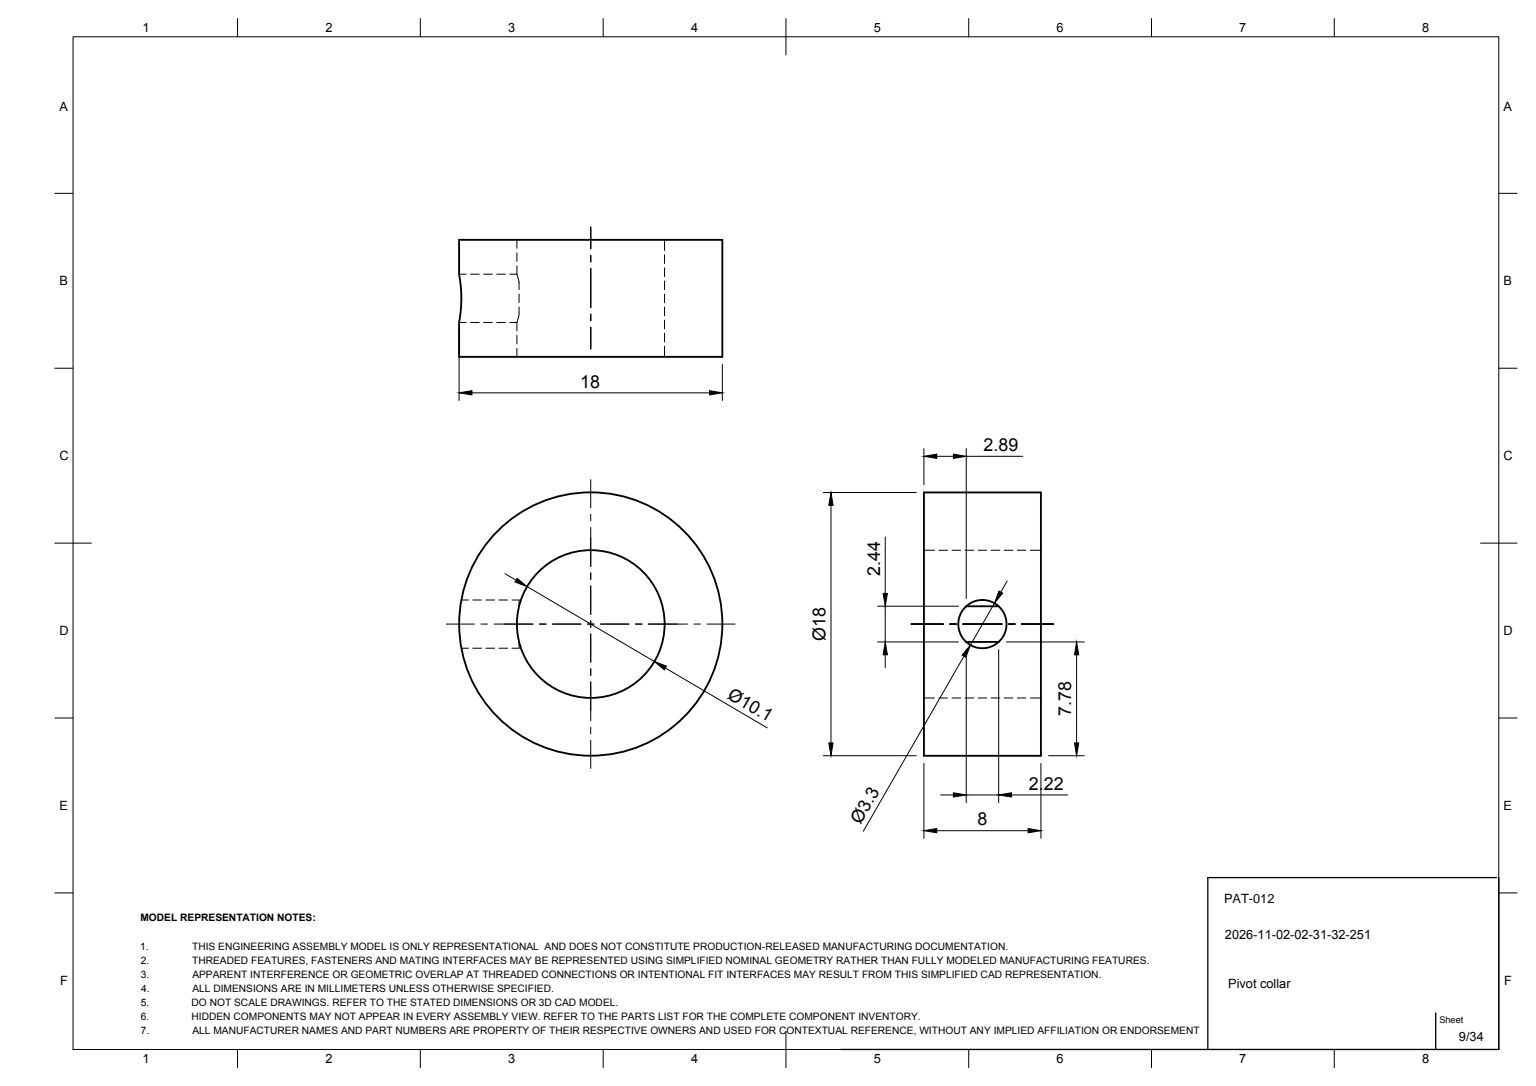
ISO-10303-21;
HEADER;
/* Generated by software containing ST-Developer
 * from STEP Tools, Inc. (www.steptools.com) 
 */

FILE_DESCRIPTION(
/* description */ ('Belt tensioner idler arm'),
/* implementation_level */ '2;1');

FILE_NAME(
/* name */ 'Pivot collar.step',
/* time_stamp */ '2026-10-28T03:22:15-07:00',
/* author */ (''),
/* organization */ (''),
/* preprocessor_version */ 'ST-DEVELOPER v20.2',
/* originating_system */ 'Autodesk Translation Framework v15.17.0.0',
/* authorisation */ '');

FILE_SCHEMA (('AUTOMOTIVE_DESIGN { 1 0 10303 214 3 1 1 }'));
ENDSEC;

DATA;
#10=MECHANICAL_DESIGN_GEOMETRIC_PRESENTATION_REPRESENTATION('',(#451),#12779);
#317=B_SPLINE_CURVE_WITH_KNOTS('',3,(#9613,#9614,#9615,#9616,#9617,#9618,
#9619,#9620,#9621,#9622,#9623,#9624,#9625,#9626),.UNSPECIFIED.,.F.,.F.,
(4,2,2,2,2,2,4),(0.618551524396292,0.626563103102765,0.689203386094988,
0.751843669087211,0.814483952079434,0.877124235071657,0.88513581377813),
 .UNSPECIFIED.);
#318=B_SPLINE_CURVE_WITH_KNOTS('',3,(#9630,#9631,#9632,#9633,#9634,#9635,
#9636,#9637),.UNSPECIFIED.,.F.,.F.,(4,2,2,4),(0.250614556362404,0.313254839354627,
0.37589512234685,0.383906701053323),.UNSPECIFIED.);
#319=B_SPLINE_CURVE_WITH_KNOTS('',3,(#9641,#9642,#9643,#9644,#9645,#9646,
#9647,#9648,#9649,#9650,#9651,#9652,#9653,#9654,#9655,#9656,#9657,#9658,
#9659,#9660,#9661,#9662,#9663,#9664,#9665,#9666),.UNSPECIFIED.,.F.,.F.,
(4,2,2,2,2,2,2,2,2,2,2,2,4),(0.,0.0623062782223143,0.124612556444629,0.186916384615149,
0.249220212785669,0.31152404095619,0.37382786912671,0.436134147349024,0.498440425571339,
0.560746703793653,0.623052982015967,0.685356810186488,0.747660638357008),
 .UNSPECIFIED.);
#320=B_SPLINE_CURVE_WITH_KNOTS('',3,(#9667,#9668,#9669,#9670,#9671,#9672,
#9673,#9674,#9675,#9676),.UNSPECIFIED.,.F.,.F.,(4,2,2,2,4),(0.747660638357008,
0.809964466527528,0.872268294698049,0.934574572920363,0.996880851142677),
 .UNSPECIFIED.);
#321=B_SPLINE_CURVE_WITH_KNOTS('',3,(#9677,#9678,#9679,#9680,#9681,#9682,
#9683,#9684),.UNSPECIFIED.,.F.,.F.,(4,2,2,4),(0.117322411671484,0.125333990377958,
0.187974273370181,0.250614556362404),.UNSPECIFIED.);
#383=SHAPE_REPRESENTATION_RELATIONSHIP('SRR','None',#12929,#417);
#417=ADVANCED_BREP_SHAPE_REPRESENTATION('',(#493),#12746);
#451=STYLED_ITEM('',(#13170),#493);
#493=MANIFOLD_SOLID_BREP('Body1',#6185);
#546=FACE_BOUND('',#1262,.T.);
#547=FACE_BOUND('',#1264,.T.);
#548=FACE_BOUND('',#1266,.T.);
#549=FACE_BOUND('',#1268,.T.);
#686=PLANE('',#6668);
#687=PLANE('',#6672);
#688=PLANE('',#6679);
#689=PLANE('',#6680);
#872=FACE_OUTER_BOUND('',#1258,.T.);
#873=FACE_OUTER_BOUND('',#1259,.T.);
#874=FACE_OUTER_BOUND('',#1260,.T.);
#875=FACE_OUTER_BOUND('',#1261,.T.);
#876=FACE_OUTER_BOUND('',#1263,.T.);
#877=FACE_OUTER_BOUND('',#1265,.T.);
#878=FACE_OUTER_BOUND('',#1267,.T.);
#1258=EDGE_LOOP('',(#4230,#4231));
#1259=EDGE_LOOP('',(#4232,#4233,#4234,#4235,#4236,#4237,#4238,#4239,#4240));
#1260=EDGE_LOOP('',(#4241,#4242));
#1261=EDGE_LOOP('',(#4243,#4244,#4245,#4246));
#1262=EDGE_LOOP('',(#4247,#4248,#4249,#4250,#4251));
#1263=EDGE_LOOP('',(#4252,#4253,#4254,#4255));
#1264=EDGE_LOOP('',(#4256,#4257));
#1265=EDGE_LOOP('',(#4258));
#1266=EDGE_LOOP('',(#4259));
#1267=EDGE_LOOP('',(#4260));
#1268=EDGE_LOOP('',(#4261));
#1755=LINE('',#9609,#2104);
#1756=LINE('',#9639,#2105);
#1757=LINE('',#9686,#2106);
#1758=LINE('',#9691,#2107);
#1759=LINE('',#9697,#2108);
#2104=VECTOR('',#7615,1.);
#2105=VECTOR('',#7622,0.165);
#2106=VECTOR('',#7625,1.);
#2107=VECTOR('',#7630,0.505);
#2108=VECTOR('',#7637,0.9);
#2429=CIRCLE('',#6669,0.165);
#2430=CIRCLE('',#6671,0.165);
#2431=CIRCLE('',#6674,0.505);
#2432=CIRCLE('',#6675,0.505);
#2433=CIRCLE('',#6677,0.9);
#2434=CIRCLE('',#6678,0.9);
#2817=VERTEX_POINT('',#9607);
#2818=VERTEX_POINT('',#9608);
#2819=VERTEX_POINT('',#9612);
#2820=VERTEX_POINT('',#9627);
#2821=VERTEX_POINT('',#9629);
#2822=VERTEX_POINT('',#9638);
#2823=VERTEX_POINT('',#9640);
#2824=VERTEX_POINT('',#9688);
#2825=VERTEX_POINT('',#9690);
#2826=VERTEX_POINT('',#9694);
#2827=VERTEX_POINT('',#9696);
#3370=EDGE_CURVE('',#2817,#2818,#1755,.T.);
#3371=EDGE_CURVE('',#2817,#2818,#2429,.T.);
#3372=EDGE_CURVE('',#2819,#2817,#317,.T.);
#3373=EDGE_CURVE('',#2820,#2819,#2430,.T.);
#3374=EDGE_CURVE('',#2821,#2820,#318,.T.);
#3375=EDGE_CURVE('',#2821,#2822,#1756,.T.);
#3376=EDGE_CURVE('',#2823,#2822,#319,.T.);
#3377=EDGE_CURVE('',#2822,#2823,#320,.T.);
#3378=EDGE_CURVE('',#2818,#2821,#321,.T.);
#3379=EDGE_CURVE('',#2820,#2819,#1757,.T.);
#3380=EDGE_CURVE('',#2824,#2824,#2431,.T.);
#3381=EDGE_CURVE('',#2824,#2825,#1758,.T.);
#3382=EDGE_CURVE('',#2825,#2825,#2432,.T.);
#3383=EDGE_CURVE('',#2826,#2826,#2433,.T.);
#3384=EDGE_CURVE('',#2826,#2827,#1759,.T.);
#3385=EDGE_CURVE('',#2827,#2827,#2434,.T.);
#4230=ORIENTED_EDGE('',*,*,#3370,.F.);
#4231=ORIENTED_EDGE('',*,*,#3371,.T.);
#4232=ORIENTED_EDGE('',*,*,#3372,.F.);
#4233=ORIENTED_EDGE('',*,*,#3373,.F.);
#4234=ORIENTED_EDGE('',*,*,#3374,.F.);
#4235=ORIENTED_EDGE('',*,*,#3375,.T.);
#4236=ORIENTED_EDGE('',*,*,#3376,.F.);
#4237=ORIENTED_EDGE('',*,*,#3377,.F.);
#4238=ORIENTED_EDGE('',*,*,#3375,.F.);
#4239=ORIENTED_EDGE('',*,*,#3378,.F.);
#4240=ORIENTED_EDGE('',*,*,#3371,.F.);
#4241=ORIENTED_EDGE('',*,*,#3379,.F.);
#4242=ORIENTED_EDGE('',*,*,#3373,.T.);
#4243=ORIENTED_EDGE('',*,*,#3380,.F.);
#4244=ORIENTED_EDGE('',*,*,#3381,.T.);
#4245=ORIENTED_EDGE('',*,*,#3382,.T.);
#4246=ORIENTED_EDGE('',*,*,#3381,.F.);
#4247=ORIENTED_EDGE('',*,*,#3378,.T.);
#4248=ORIENTED_EDGE('',*,*,#3374,.T.);
#4249=ORIENTED_EDGE('',*,*,#3379,.T.);
#4250=ORIENTED_EDGE('',*,*,#3372,.T.);
#4251=ORIENTED_EDGE('',*,*,#3370,.T.);
#4252=ORIENTED_EDGE('',*,*,#3383,.F.);
#4253=ORIENTED_EDGE('',*,*,#3384,.T.);
#4254=ORIENTED_EDGE('',*,*,#3385,.T.);
#4255=ORIENTED_EDGE('',*,*,#3384,.F.);
#4256=ORIENTED_EDGE('',*,*,#3376,.T.);
#4257=ORIENTED_EDGE('',*,*,#3377,.T.);
#4258=ORIENTED_EDGE('',*,*,#3383,.T.);
#4259=ORIENTED_EDGE('',*,*,#3380,.T.);
#4260=ORIENTED_EDGE('',*,*,#3385,.F.);
#4261=ORIENTED_EDGE('',*,*,#3382,.F.);
#5674=CYLINDRICAL_SURFACE('',#6670,0.165);
#5675=CYLINDRICAL_SURFACE('',#6673,0.505);
#5676=CYLINDRICAL_SURFACE('',#6676,0.9);
#5849=ADVANCED_FACE('',(#872),#686,.T.);
#5850=ADVANCED_FACE('',(#873),#5674,.F.);
#5851=ADVANCED_FACE('',(#874),#687,.T.);
#5852=ADVANCED_FACE('',(#875,#546),#5675,.F.);
#5853=ADVANCED_FACE('',(#876,#547),#5676,.T.);
#5854=ADVANCED_FACE('',(#877,#548),#688,.T.);
#5855=ADVANCED_FACE('',(#878,#549),#689,.F.);
#6185=CLOSED_SHELL('',(#5849,#5850,#5851,#5852,#5853,#5854,#5855));
#6667=AXIS2_PLACEMENT_3D('',#9605,#7611,#7612);
#6668=AXIS2_PLACEMENT_3D('',#9606,#7613,#7614);
#6669=AXIS2_PLACEMENT_3D('',#9610,#7616,#7617);
#6670=AXIS2_PLACEMENT_3D('',#9611,#7618,#7619);
#6671=AXIS2_PLACEMENT_3D('',#9628,#7620,#7621);
#6672=AXIS2_PLACEMENT_3D('',#9685,#7623,#7624);
#6673=AXIS2_PLACEMENT_3D('',#9687,#7626,#7627);
#6674=AXIS2_PLACEMENT_3D('',#9689,#7628,#7629);
#6675=AXIS2_PLACEMENT_3D('',#9692,#7631,#7632);
#6676=AXIS2_PLACEMENT_3D('',#9693,#7633,#7634);
#6677=AXIS2_PLACEMENT_3D('',#9695,#7635,#7636);
#6678=AXIS2_PLACEMENT_3D('',#9698,#7638,#7639);
#6679=AXIS2_PLACEMENT_3D('',#9699,#7640,#7641);
#6680=AXIS2_PLACEMENT_3D('',#9700,#7642,#7643);
#7611=DIRECTION('axis',(0.,0.,1.));
#7612=DIRECTION('refdir',(1.,0.,0.));
#7613=DIRECTION('center_axis',(1.,0.,0.));
#7614=DIRECTION('ref_axis',(0.,0.,-1.));
#7615=DIRECTION('',(0.,0.,1.));
#7616=DIRECTION('center_axis',(1.,0.,0.));
#7617=DIRECTION('ref_axis',(0.,0.,-1.));
#7618=DIRECTION('center_axis',(1.,0.,0.));
#7619=DIRECTION('ref_axis',(0.,0.,-1.));
#7620=DIRECTION('center_axis',(1.,0.,0.));
#7621=DIRECTION('ref_axis',(0.,0.,-1.));
#7622=DIRECTION('',(1.,0.,0.));
#7623=DIRECTION('center_axis',(1.,0.,0.));
#7624=DIRECTION('ref_axis',(0.,0.,-1.));
#7625=DIRECTION('',(0.,0.,-1.));
#7626=DIRECTION('center_axis',(0.,0.,1.));
#7627=DIRECTION('ref_axis',(1.,0.,0.));
#7628=DIRECTION('center_axis',(0.,0.,-1.));
#7629=DIRECTION('ref_axis',(1.,0.,0.));
#7630=DIRECTION('',(0.,0.,-1.));
#7631=DIRECTION('center_axis',(0.,0.,-1.));
#7632=DIRECTION('ref_axis',(1.,0.,0.));
#7633=DIRECTION('center_axis',(0.,0.,1.));
#7634=DIRECTION('ref_axis',(1.,0.,0.));
#7635=DIRECTION('center_axis',(0.,0.,1.));
#7636=DIRECTION('ref_axis',(1.,0.,0.));
#7637=DIRECTION('',(0.,0.,-1.));
#7638=DIRECTION('center_axis',(0.,0.,1.));
#7639=DIRECTION('ref_axis',(1.,0.,0.));
#7640=DIRECTION('center_axis',(0.,0.,1.));
#7641=DIRECTION('ref_axis',(1.,0.,0.));
#7642=DIRECTION('center_axis',(0.,0.,1.));
#7643=DIRECTION('ref_axis',(1.,0.,0.));
#9605=CARTESIAN_POINT('',(0.,0.,0.));
#9606=CARTESIAN_POINT('Origin',(0.49,0.,6.35));
#9607=CARTESIAN_POINT('',(0.49,0.122167917228706,6.2390946349359));
#9608=CARTESIAN_POINT('',(0.49,0.122167917228706,6.46090536506409));
#9609=CARTESIAN_POINT('',(0.49,0.122167917228706,5.95));
#9610=CARTESIAN_POINT('Origin',(0.49,0.,6.35));
#9611=CARTESIAN_POINT('Origin',(0.49,0.,6.35));
#9612=CARTESIAN_POINT('',(0.49,-0.122167917228706,6.2390946349359));
#9613=CARTESIAN_POINT('Ctrl Pts',(0.49,-0.122167917228706,6.2390946349359));
#9614=CARTESIAN_POINT('Ctrl Pts',(0.490448531679987,-0.120368913626295,
6.23711294069536));
#9615=CARTESIAN_POINT('Ctrl Pts',(0.490895245371684,-0.118534896565231,
6.23518965877367));
#9616=CARTESIAN_POINT('Ctrl Pts',(0.494795015531646,-0.102111993019358,
6.2187667552278));
#9617=CARTESIAN_POINT('Ctrl Pts',(0.498442514607595,-0.0836597150224318,
6.20609154388858));
#9618=CARTESIAN_POINT('Ctrl Pts',(0.50357781976106,-0.0430495960471596,
6.18920409039234));
#9619=CARTESIAN_POINT('Ctrl Pts',(0.505,-0.020880094330741,6.185));
#9620=CARTESIAN_POINT('Ctrl Pts',(0.505,0.020880094330741,6.185));
#9621=CARTESIAN_POINT('Ctrl Pts',(0.50357781976106,0.0430495960471596,6.18920409039234));
#9622=CARTESIAN_POINT('Ctrl Pts',(0.498442514607595,0.0836597150224318,
6.20609154388858));
#9623=CARTESIAN_POINT('Ctrl Pts',(0.494795015531646,0.102111993019358,6.2187667552278));
#9624=CARTESIAN_POINT('Ctrl Pts',(0.490895245371685,0.118534896565231,6.23518965877367));
#9625=CARTESIAN_POINT('Ctrl Pts',(0.490448531679987,0.120368913626295,6.23711294069536));
#9626=CARTESIAN_POINT('Ctrl Pts',(0.49,0.122167917228706,6.2390946349359));
#9627=CARTESIAN_POINT('',(0.49,-0.122167917228706,6.46090536506409));
#9628=CARTESIAN_POINT('Origin',(0.49,0.,6.35));
#9629=CARTESIAN_POINT('',(0.505,4.88772620902458E-17,6.515));
#9630=CARTESIAN_POINT('Ctrl Pts',(0.505,1.2490009027033E-16,6.515));
#9631=CARTESIAN_POINT('Ctrl Pts',(0.505,-0.0208800943307409,6.515));
#9632=CARTESIAN_POINT('Ctrl Pts',(0.50357781976106,-0.0430495960471596,
6.51079590960766));
#9633=CARTESIAN_POINT('Ctrl Pts',(0.498442514607595,-0.0836597150224318,
6.49390845611142));
#9634=CARTESIAN_POINT('Ctrl Pts',(0.494795015531646,-0.102111993019358,
6.4812332447722));
#9635=CARTESIAN_POINT('Ctrl Pts',(0.490895245371684,-0.118534896565231,
6.46481034122633));
#9636=CARTESIAN_POINT('Ctrl Pts',(0.490448531679987,-0.120368913626296,
6.46288705930464));
#9637=CARTESIAN_POINT('Ctrl Pts',(0.49,-0.122167917228706,6.46090536506409));
#9638=CARTESIAN_POINT('',(0.9,-2.02066721859313E-17,6.515));
#9639=CARTESIAN_POINT('',(0.49,-2.02066721859313E-17,6.515));
#9640=CARTESIAN_POINT('',(0.884745726183518,0.165,6.35));
#9641=CARTESIAN_POINT('Ctrl Pts',(0.884745726183518,0.165,6.35));
#9642=CARTESIAN_POINT('Ctrl Pts',(0.884745726183518,0.165,6.32923124059256));
#9643=CARTESIAN_POINT('Ctrl Pts',(0.885552759505264,0.160839719007584,6.30711110492665));
#9644=CARTESIAN_POINT('Ctrl Pts',(0.888448648150043,0.14398647021669,6.26647293736623));
#9645=CARTESIAN_POINT('Ctrl Pts',(0.890493604851638,0.131295993814186,6.24795075602263));
#9646=CARTESIAN_POINT('Ctrl Pts',(0.89431723432394,0.102049819008125,6.21870458121656));
#9647=CARTESIAN_POINT('Ctrl Pts',(0.896347088899543,0.0835273920906821,
6.20601365401642));
#9648=CARTESIAN_POINT('Ctrl Pts',(0.899208271860583,0.0428883760934128,
6.18916007816136));
#9649=CARTESIAN_POINT('Ctrl Pts',(0.9,0.0207679427235068,6.185));
#9650=CARTESIAN_POINT('Ctrl Pts',(0.9,-0.0207679427235068,6.185));
#9651=CARTESIAN_POINT('Ctrl Pts',(0.899208271860583,-0.0428883760934128,
6.18916007816136));
#9652=CARTESIAN_POINT('Ctrl Pts',(0.896347088899543,-0.0835273920906821,
6.20601365401642));
#9653=CARTESIAN_POINT('Ctrl Pts',(0.89431723432394,-0.102049819008125,6.21870458121656));
#9654=CARTESIAN_POINT('Ctrl Pts',(0.890493604851638,-0.131295993814186,
6.24795075602263));
#9655=CARTESIAN_POINT('Ctrl Pts',(0.888448648150043,-0.14398647021669,6.26647293736623));
#9656=CARTESIAN_POINT('Ctrl Pts',(0.885552759505264,-0.160839719007584,
6.30711110492665));
#9657=CARTESIAN_POINT('Ctrl Pts',(0.884745726183518,-0.165,6.32923124059256));
#9658=CARTESIAN_POINT('Ctrl Pts',(0.884745726183518,-0.165,6.37076875940744));
#9659=CARTESIAN_POINT('Ctrl Pts',(0.885552759505264,-0.160839719007584,
6.39288889507334));
#9660=CARTESIAN_POINT('Ctrl Pts',(0.888448648150043,-0.14398647021669,6.43352706263377));
#9661=CARTESIAN_POINT('Ctrl Pts',(0.890493604851638,-0.131295993814186,
6.45204924397737));
#9662=CARTESIAN_POINT('Ctrl Pts',(0.89431723432394,-0.102049819008125,6.48129541878344));
#9663=CARTESIAN_POINT('Ctrl Pts',(0.896347088899543,-0.0835273920906822,
6.49398634598358));
#9664=CARTESIAN_POINT('Ctrl Pts',(0.899208271860583,-0.0428883760934128,
6.51083992183864));
#9665=CARTESIAN_POINT('Ctrl Pts',(0.9,-0.0207679427235068,6.515));
#9666=CARTESIAN_POINT('Ctrl Pts',(0.9,0.,6.515));
#9667=CARTESIAN_POINT('Ctrl Pts',(0.9,-4.16333634234434E-17,6.515));
#9668=CARTESIAN_POINT('Ctrl Pts',(0.9,0.0207679427235068,6.515));
#9669=CARTESIAN_POINT('Ctrl Pts',(0.899208271860583,0.0428883760934128,
6.51083992183864));
#9670=CARTESIAN_POINT('Ctrl Pts',(0.896347088899543,0.0835273920906821,
6.49398634598358));
#9671=CARTESIAN_POINT('Ctrl Pts',(0.89431723432394,0.102049819008125,6.48129541878344));
#9672=CARTESIAN_POINT('Ctrl Pts',(0.890493604851638,0.131295993814186,6.45204924397737));
#9673=CARTESIAN_POINT('Ctrl Pts',(0.888448648150043,0.14398647021669,6.43352706263377));
#9674=CARTESIAN_POINT('Ctrl Pts',(0.885552759505264,0.160839719007584,6.39288889507334));
#9675=CARTESIAN_POINT('Ctrl Pts',(0.884745726183518,0.165,6.37076875940744));
#9676=CARTESIAN_POINT('Ctrl Pts',(0.884745726183518,0.165,6.35));
#9677=CARTESIAN_POINT('Ctrl Pts',(0.49,0.122167917228706,6.46090536506409));
#9678=CARTESIAN_POINT('Ctrl Pts',(0.490448531679987,0.120368913626296,6.46288705930464));
#9679=CARTESIAN_POINT('Ctrl Pts',(0.490895245371684,0.118534896565231,6.46481034122633));
#9680=CARTESIAN_POINT('Ctrl Pts',(0.494795015531646,0.102111993019358,6.4812332447722));
#9681=CARTESIAN_POINT('Ctrl Pts',(0.498442514607595,0.0836597150224318,
6.49390845611142));
#9682=CARTESIAN_POINT('Ctrl Pts',(0.50357781976106,0.0430495960471596,6.51079590960766));
#9683=CARTESIAN_POINT('Ctrl Pts',(0.505,0.0208800943307409,6.515));
#9684=CARTESIAN_POINT('Ctrl Pts',(0.505,-1.11022302462516E-16,6.515));
#9685=CARTESIAN_POINT('Origin',(0.49,0.,6.35));
#9686=CARTESIAN_POINT('',(0.49,-0.122167917228706,5.95));
#9687=CARTESIAN_POINT('Origin',(0.,0.,5.95));
#9688=CARTESIAN_POINT('',(-0.505,-6.18446633569413E-17,6.75));
#9689=CARTESIAN_POINT('Origin',(0.,0.,6.75));
#9690=CARTESIAN_POINT('',(-0.505,-6.18446633569413E-17,5.95));
#9691=CARTESIAN_POINT('',(-0.505,-6.18446633569413E-17,5.95));
#9692=CARTESIAN_POINT('Origin',(0.,0.,5.95));
#9693=CARTESIAN_POINT('Origin',(0.,0.,5.95));
#9694=CARTESIAN_POINT('',(-0.9,-1.10218211923262E-16,6.75));
#9695=CARTESIAN_POINT('Origin',(0.,0.,6.75));
#9696=CARTESIAN_POINT('',(-0.9,-1.10218211923262E-16,5.95));
#9697=CARTESIAN_POINT('',(-0.9,-1.10218211923262E-16,5.95));
#9698=CARTESIAN_POINT('Origin',(0.,0.,5.95));
#9699=CARTESIAN_POINT('Origin',(0.,0.,6.75));
#9700=CARTESIAN_POINT('Origin',(0.,0.,5.95));
#12706=UNCERTAINTY_MEASURE_WITH_UNIT(LENGTH_MEASURE(0.001),#12780,
'DISTANCE_ACCURACY_VALUE',
'Maximum model space distance between geometric entities at asserted c
onnectivities');
#12739=UNCERTAINTY_MEASURE_WITH_UNIT(LENGTH_MEASURE(0.001),#12780,
'DISTANCE_ACCURACY_VALUE',
'Maximum model space distance between geometric entities at asserted c
onnectivities');
#12746=(
GEOMETRIC_REPRESENTATION_CONTEXT(3)
GLOBAL_UNCERTAINTY_ASSIGNED_CONTEXT((#12706))
GLOBAL_UNIT_ASSIGNED_CONTEXT((#12780,#12782,#12783))
REPRESENTATION_CONTEXT('','3D')
);
#12779=(
GEOMETRIC_REPRESENTATION_CONTEXT(3)
GLOBAL_UNCERTAINTY_ASSIGNED_CONTEXT((#12739))
GLOBAL_UNIT_ASSIGNED_CONTEXT((#12780,#12782,#12783))
REPRESENTATION_CONTEXT('','3D')
);
#12780=(
LENGTH_UNIT()
NAMED_UNIT(*)
SI_UNIT(.CENTI.,.METRE.)
);
#12782=(
NAMED_UNIT(*)
PLANE_ANGLE_UNIT()
SI_UNIT($,.RADIAN.)
);
#12783=(
NAMED_UNIT(*)
SI_UNIT($,.STERADIAN.)
SOLID_ANGLE_UNIT()
);
#12790=SHAPE_DEFINITION_REPRESENTATION(#12829,#12929);
#12829=PRODUCT_DEFINITION_SHAPE('',$,#12969);
#12929=SHAPE_REPRESENTATION('',(#6667),#12746);
#12962=PRODUCT_DEFINITION_CONTEXT('part definition',#13081,'design');
#12969=PRODUCT_DEFINITION('Pivot collar','Pivot collar',#13008,#12962);
#13008=PRODUCT_DEFINITION_FORMATION('',$,#13089);
#13081=APPLICATION_CONTEXT(
'Core Data for Automotive Mechanical Design Process');
#13082=PRODUCT_CONTEXT('part definition',#13081,'mechanical');
#13089=PRODUCT('Pivot collar','Pivot collar','Pivot collar',(#13082));
#13164=COLOUR_RGB('Light Blue',0.38,0.62,0.78);
#13165=FILL_AREA_STYLE_COLOUR('',#13164);
#13166=FILL_AREA_STYLE('',(#13165));
#13167=SURFACE_STYLE_FILL_AREA(#13166);
#13168=SURFACE_SIDE_STYLE('',(#13167));
#13169=SURFACE_STYLE_USAGE(.BOTH.,#13168);
#13170=PRESENTATION_STYLE_ASSIGNMENT((#13169));
ENDSEC;
END-ISO-10303-21;
